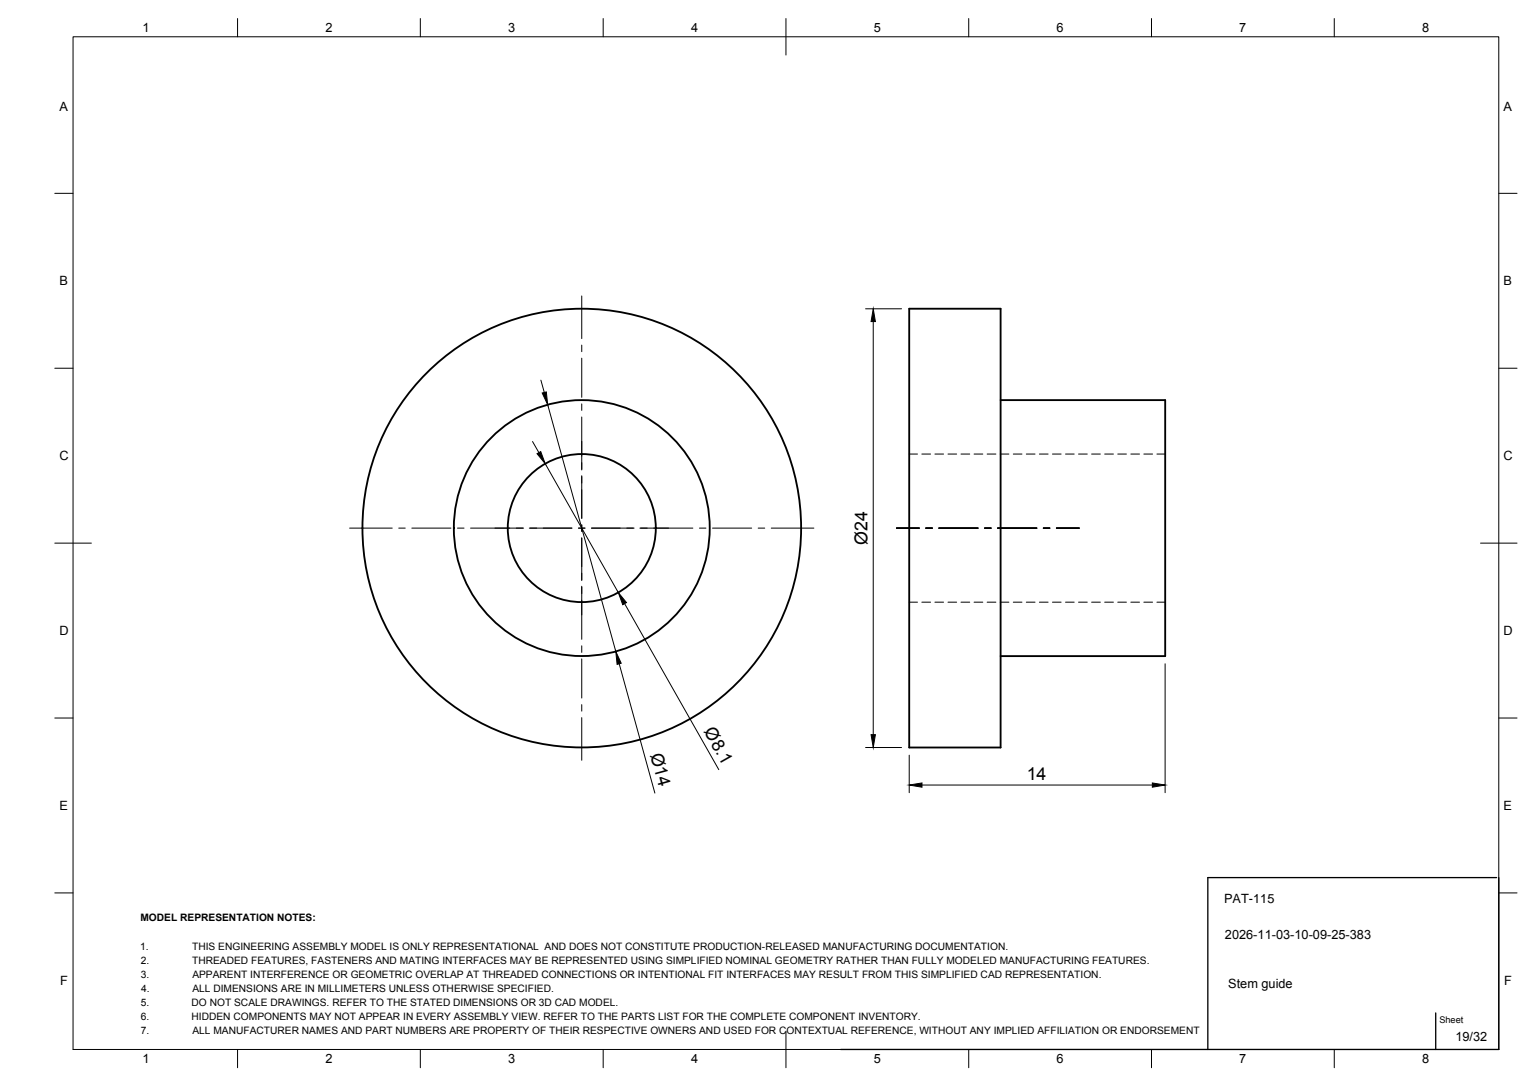
ISO-10303-21;
HEADER;
/* Generated by software containing ST-Developer
 * from STEP Tools, Inc. (www.steptools.com) 
 */

FILE_DESCRIPTION(
/* description */ ('Union bypass pipe loop'),
/* implementation_level */ '2;1');

FILE_NAME(
/* name */ 'Stem guide.step',
/* time_stamp */ '2026-10-27T21:00:29-07:00',
/* author */ (''),
/* organization */ (''),
/* preprocessor_version */ 'ST-DEVELOPER v20.2',
/* originating_system */ 'Autodesk Translation Framework v15.17.0.0',
/* authorisation */ '');

FILE_SCHEMA (('AUTOMOTIVE_DESIGN { 1 0 10303 214 3 1 1 }'));
ENDSEC;

DATA;
#10=MECHANICAL_DESIGN_GEOMETRIC_PRESENTATION_REPRESENTATION('',(#448),#10095);
#384=SHAPE_REPRESENTATION_RELATIONSHIP('SRR','None',#10253,#416);
#416=ADVANCED_BREP_SHAPE_REPRESENTATION('',(#480),#10065);
#448=STYLED_ITEM('',(#10493),#480);
#480=MANIFOLD_SOLID_BREP('Body1',#5519);
#547=FACE_BOUND('',#1262,.T.);
#548=FACE_BOUND('',#1265,.T.);
#549=FACE_BOUND('',#1269,.T.);
#668=PLANE('',#6022);
#669=PLANE('',#6027);
#670=PLANE('',#6033);
#893=FACE_OUTER_BOUND('',#1261,.T.);
#894=FACE_OUTER_BOUND('',#1263,.T.);
#895=FACE_OUTER_BOUND('',#1264,.T.);
#896=FACE_OUTER_BOUND('',#1266,.T.);
#897=FACE_OUTER_BOUND('',#1267,.T.);
#898=FACE_OUTER_BOUND('',#1268,.T.);
#1261=EDGE_LOOP('',(#4006));
#1262=EDGE_LOOP('',(#4007));
#1263=EDGE_LOOP('',(#4008,#4009,#4010,#4011));
#1264=EDGE_LOOP('',(#4012));
#1265=EDGE_LOOP('',(#4013));
#1266=EDGE_LOOP('',(#4014,#4015,#4016,#4017));
#1267=EDGE_LOOP('',(#4018,#4019,#4020,#4021));
#1268=EDGE_LOOP('',(#4022));
#1269=EDGE_LOOP('',(#4023));
#1705=LINE('',#8720,#2081);
#1706=LINE('',#8726,#2082);
#1707=LINE('',#8730,#2083);
#2081=VECTOR('',#6945,1.2);
#2082=VECTOR('',#6952,0.405);
#2083=VECTOR('',#6957,0.7);
#2427=CIRCLE('',#6023,1.2);
#2428=CIRCLE('',#6024,0.7);
#2429=CIRCLE('',#6026,1.2);
#2430=CIRCLE('',#6028,0.405);
#2431=CIRCLE('',#6030,0.405);
#2432=CIRCLE('',#6032,0.7);
#2720=VERTEX_POINT('',#8713);
#2721=VERTEX_POINT('',#8715);
#2722=VERTEX_POINT('',#8718);
#2723=VERTEX_POINT('',#8722);
#2724=VERTEX_POINT('',#8725);
#2725=VERTEX_POINT('',#8729);
#3201=EDGE_CURVE('',#2720,#2720,#2427,.T.);
#3202=EDGE_CURVE('',#2721,#2721,#2428,.T.);
#3203=EDGE_CURVE('',#2722,#2722,#2429,.T.);
#3204=EDGE_CURVE('',#2722,#2720,#1705,.T.);
#3205=EDGE_CURVE('',#2723,#2723,#2430,.T.);
#3206=EDGE_CURVE('',#2723,#2724,#1706,.T.);
#3207=EDGE_CURVE('',#2724,#2724,#2431,.T.);
#3208=EDGE_CURVE('',#2721,#2725,#1707,.T.);
#3209=EDGE_CURVE('',#2725,#2725,#2432,.T.);
#4006=ORIENTED_EDGE('',*,*,#3201,.F.);
#4007=ORIENTED_EDGE('',*,*,#3202,.T.);
#4008=ORIENTED_EDGE('',*,*,#3203,.F.);
#4009=ORIENTED_EDGE('',*,*,#3204,.T.);
#4010=ORIENTED_EDGE('',*,*,#3201,.T.);
#4011=ORIENTED_EDGE('',*,*,#3204,.F.);
#4012=ORIENTED_EDGE('',*,*,#3203,.T.);
#4013=ORIENTED_EDGE('',*,*,#3205,.T.);
#4014=ORIENTED_EDGE('',*,*,#3205,.F.);
#4015=ORIENTED_EDGE('',*,*,#3206,.T.);
#4016=ORIENTED_EDGE('',*,*,#3207,.T.);
#4017=ORIENTED_EDGE('',*,*,#3206,.F.);
#4018=ORIENTED_EDGE('',*,*,#3202,.F.);
#4019=ORIENTED_EDGE('',*,*,#3208,.T.);
#4020=ORIENTED_EDGE('',*,*,#3209,.T.);
#4021=ORIENTED_EDGE('',*,*,#3208,.F.);
#4022=ORIENTED_EDGE('',*,*,#3209,.F.);
#4023=ORIENTED_EDGE('',*,*,#3207,.F.);
#5103=CYLINDRICAL_SURFACE('',#6025,1.2);
#5104=CYLINDRICAL_SURFACE('',#6029,0.405);
#5105=CYLINDRICAL_SURFACE('',#6031,0.7);
#5242=ADVANCED_FACE('',(#893,#547),#668,.F.);
#5243=ADVANCED_FACE('',(#894),#5103,.T.);
#5244=ADVANCED_FACE('',(#895,#548),#669,.T.);
#5245=ADVANCED_FACE('',(#896),#5104,.F.);
#5246=ADVANCED_FACE('',(#897),#5105,.T.);
#5247=ADVANCED_FACE('',(#898,#549),#670,.F.);
#5519=CLOSED_SHELL('',(#5242,#5243,#5244,#5245,#5246,#5247));
#6021=AXIS2_PLACEMENT_3D('',#8711,#6933,#6934);
#6022=AXIS2_PLACEMENT_3D('',#8712,#6935,#6936);
#6023=AXIS2_PLACEMENT_3D('',#8714,#6937,#6938);
#6024=AXIS2_PLACEMENT_3D('',#8716,#6939,#6940);
#6025=AXIS2_PLACEMENT_3D('',#8717,#6941,#6942);
#6026=AXIS2_PLACEMENT_3D('',#8719,#6943,#6944);
#6027=AXIS2_PLACEMENT_3D('',#8721,#6946,#6947);
#6028=AXIS2_PLACEMENT_3D('',#8723,#6948,#6949);
#6029=AXIS2_PLACEMENT_3D('',#8724,#6950,#6951);
#6030=AXIS2_PLACEMENT_3D('',#8727,#6953,#6954);
#6031=AXIS2_PLACEMENT_3D('',#8728,#6955,#6956);
#6032=AXIS2_PLACEMENT_3D('',#8731,#6958,#6959);
#6033=AXIS2_PLACEMENT_3D('',#8732,#6960,#6961);
#6933=DIRECTION('axis',(0.,0.,1.));
#6934=DIRECTION('refdir',(1.,0.,0.));
#6935=DIRECTION('center_axis',(0.,0.,1.));
#6936=DIRECTION('ref_axis',(1.,0.,0.));
#6937=DIRECTION('center_axis',(0.,0.,1.));
#6938=DIRECTION('ref_axis',(1.,0.,0.));
#6939=DIRECTION('center_axis',(0.,0.,1.));
#6940=DIRECTION('ref_axis',(1.,0.,0.));
#6941=DIRECTION('center_axis',(0.,0.,1.));
#6942=DIRECTION('ref_axis',(1.,0.,0.));
#6943=DIRECTION('center_axis',(0.,0.,1.));
#6944=DIRECTION('ref_axis',(1.,0.,0.));
#6945=DIRECTION('',(0.,0.,-1.));
#6946=DIRECTION('center_axis',(0.,0.,1.));
#6947=DIRECTION('ref_axis',(1.,0.,0.));
#6948=DIRECTION('center_axis',(0.,0.,-1.));
#6949=DIRECTION('ref_axis',(1.,0.,0.));
#6950=DIRECTION('center_axis',(0.,0.,1.));
#6951=DIRECTION('ref_axis',(1.,0.,0.));
#6952=DIRECTION('',(0.,0.,-1.));
#6953=DIRECTION('center_axis',(0.,0.,-1.));
#6954=DIRECTION('ref_axis',(1.,0.,0.));
#6955=DIRECTION('center_axis',(0.,0.,1.));
#6956=DIRECTION('ref_axis',(1.,0.,0.));
#6957=DIRECTION('',(0.,0.,-1.));
#6958=DIRECTION('center_axis',(0.,0.,1.));
#6959=DIRECTION('ref_axis',(1.,0.,0.));
#6960=DIRECTION('center_axis',(0.,0.,1.));
#6961=DIRECTION('ref_axis',(1.,0.,0.));
#8711=CARTESIAN_POINT('',(0.,0.,0.));
#8712=CARTESIAN_POINT('Origin',(0.,0.,7.5));
#8713=CARTESIAN_POINT('',(-1.2,-1.46957615897682E-16,7.5));
#8714=CARTESIAN_POINT('Origin',(0.,0.,7.5));
#8715=CARTESIAN_POINT('',(-0.7,-8.57252759403147E-17,7.5));
#8716=CARTESIAN_POINT('Origin',(0.,0.,7.5));
#8717=CARTESIAN_POINT('Origin',(0.,0.,7.5));
#8718=CARTESIAN_POINT('',(-1.2,-1.46957615897682E-16,8.));
#8719=CARTESIAN_POINT('Origin',(0.,0.,8.));
#8720=CARTESIAN_POINT('',(-1.2,-1.46957615897682E-16,7.5));
#8721=CARTESIAN_POINT('Origin',(0.,0.,8.));
#8722=CARTESIAN_POINT('',(-0.405,-4.95981953654678E-17,8.));
#8723=CARTESIAN_POINT('Origin',(0.,0.,8.));
#8724=CARTESIAN_POINT('Origin',(0.,0.,6.6));
#8725=CARTESIAN_POINT('',(-0.405,-4.95981953654678E-17,6.6));
#8726=CARTESIAN_POINT('',(-0.405,-4.95981953654678E-17,6.6));
#8727=CARTESIAN_POINT('Origin',(0.,0.,6.6));
#8728=CARTESIAN_POINT('Origin',(0.,0.,6.6));
#8729=CARTESIAN_POINT('',(-0.7,-8.57252759403147E-17,6.6));
#8730=CARTESIAN_POINT('',(-0.7,-8.57252759403147E-17,6.6));
#8731=CARTESIAN_POINT('Origin',(0.,0.,6.6));
#8732=CARTESIAN_POINT('Origin',(0.,0.,6.6));
#10028=UNCERTAINTY_MEASURE_WITH_UNIT(LENGTH_MEASURE(0.001),#10096,
'DISTANCE_ACCURACY_VALUE',
'Maximum model space distance between geometric entities at asserted c
onnectivities');
#10058=UNCERTAINTY_MEASURE_WITH_UNIT(LENGTH_MEASURE(0.001),#10096,
'DISTANCE_ACCURACY_VALUE',
'Maximum model space distance between geometric entities at asserted c
onnectivities');
#10065=(
GEOMETRIC_REPRESENTATION_CONTEXT(3)
GLOBAL_UNCERTAINTY_ASSIGNED_CONTEXT((#10028))
GLOBAL_UNIT_ASSIGNED_CONTEXT((#10096,#10098,#10099))
REPRESENTATION_CONTEXT('','3D')
);
#10095=(
GEOMETRIC_REPRESENTATION_CONTEXT(3)
GLOBAL_UNCERTAINTY_ASSIGNED_CONTEXT((#10058))
GLOBAL_UNIT_ASSIGNED_CONTEXT((#10096,#10098,#10099))
REPRESENTATION_CONTEXT('','3D')
);
#10096=(
LENGTH_UNIT()
NAMED_UNIT(*)
SI_UNIT(.CENTI.,.METRE.)
);
#10098=(
NAMED_UNIT(*)
PLANE_ANGLE_UNIT()
SI_UNIT($,.RADIAN.)
);
#10099=(
NAMED_UNIT(*)
SI_UNIT($,.STERADIAN.)
SOLID_ANGLE_UNIT()
);
#10106=SHAPE_DEFINITION_REPRESENTATION(#10142,#10253);
#10142=PRODUCT_DEFINITION_SHAPE('',$,#10290);
#10253=SHAPE_REPRESENTATION('',(#6021),#10065);
#10283=PRODUCT_DEFINITION_CONTEXT('part definition',#10393,'design');
#10290=PRODUCT_DEFINITION('Stem guide','Stem guide',#10326,#10283);
#10326=PRODUCT_DEFINITION_FORMATION('',$,#10401);
#10393=APPLICATION_CONTEXT(
'Core Data for Automotive Mechanical Design Process');
#10394=PRODUCT_CONTEXT('part definition',#10393,'mechanical');
#10401=PRODUCT('Stem guide','Stem guide','Stem guide',(#10394));
#10487=COLOUR_RGB('Sky Blue',0.24,0.69,0.87);
#10488=FILL_AREA_STYLE_COLOUR('',#10487);
#10489=FILL_AREA_STYLE('',(#10488));
#10490=SURFACE_STYLE_FILL_AREA(#10489);
#10491=SURFACE_SIDE_STYLE('',(#10490));
#10492=SURFACE_STYLE_USAGE(.BOTH.,#10491);
#10493=PRESENTATION_STYLE_ASSIGNMENT((#10492));
ENDSEC;
END-ISO-10303-21;
